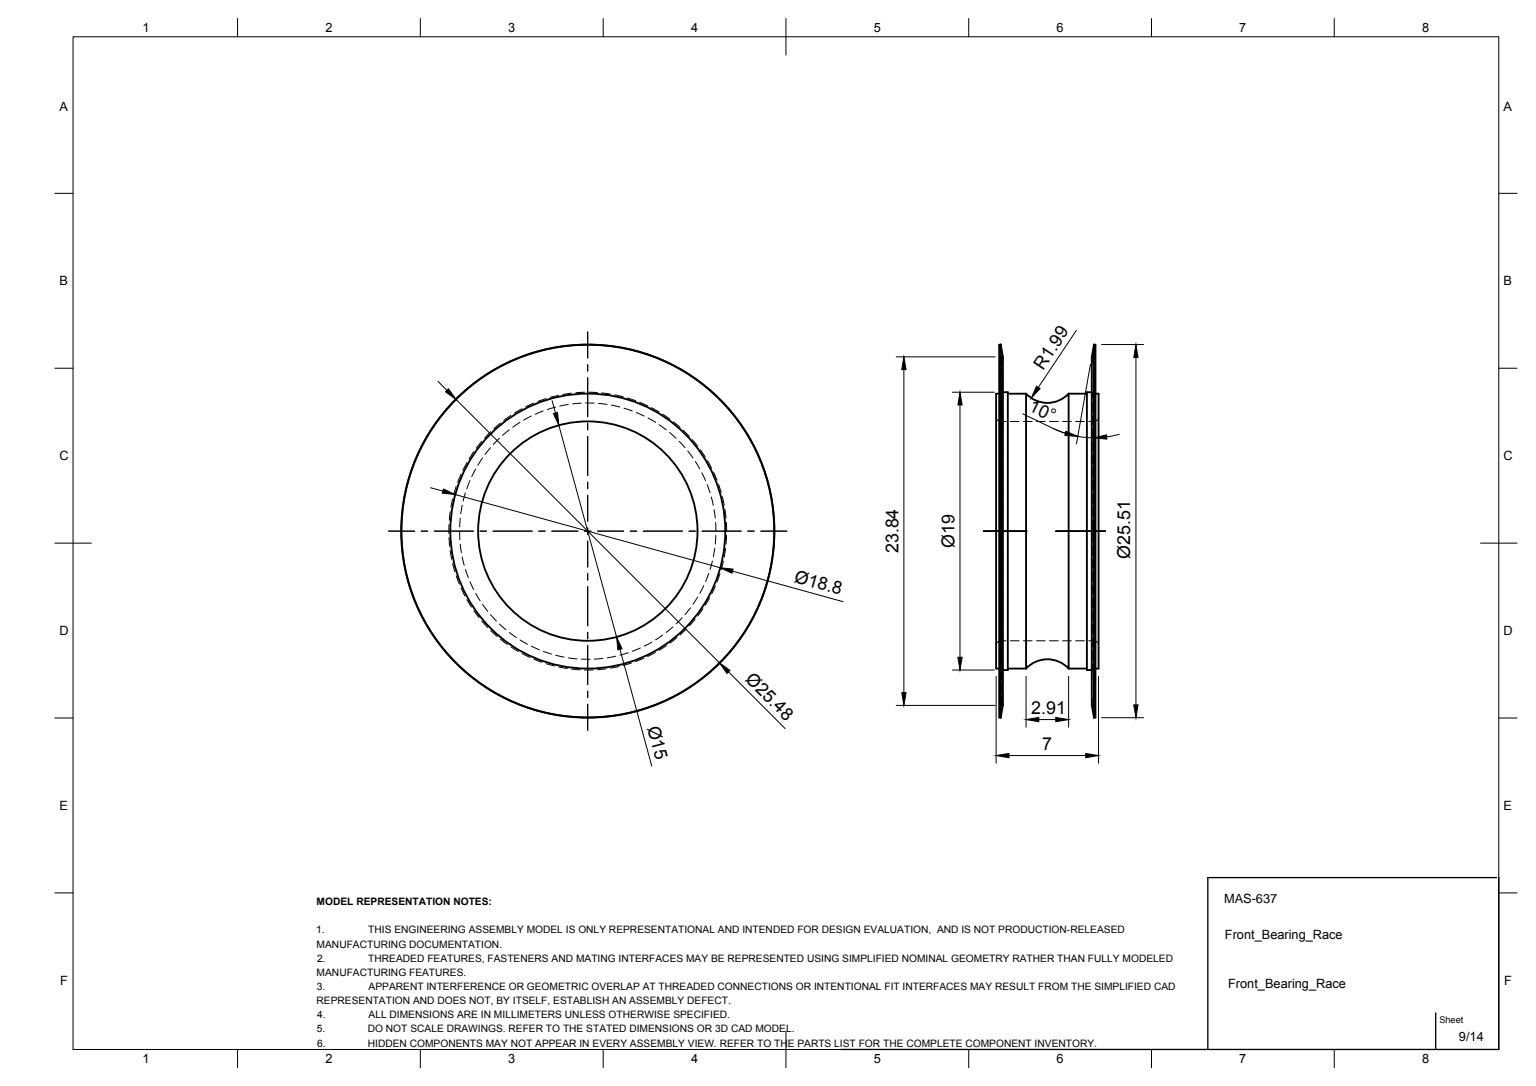
ISO-10303-21;
HEADER;
FILE_DESCRIPTION((''),'2;1');
FILE_NAME('Front_Bearing_Race.step','2026-10-09T10:11:57-07:00',(''),(''),'','','');
FILE_SCHEMA (('AUTOMOTIVE_DESIGN { 1 0 10303 214 3 1 1 }'));
ENDSEC;
DATA;
#10=MECHANICAL_DESIGN_GEOMETRIC_PRESENTATION_REPRESENTATION('',(#132),#13510);
#102=SHAPE_REPRESENTATION_RELATIONSHIP('SRR','None',#13572,#117) ;
#117=ADVANCED_BREP_SHAPE_REPRESENTATION('',(#164),#13504) ;
#132=STYLED_ITEM('',(#13650),#164) ;
#164=MANIFOLD_SOLID_BREP('Body1',#7381) ;
#246=FACE_BOUND('',#1504,.T.) ;
#247=FACE_BOUND('',#1515,.T.) ;
#248=FACE_BOUND('',#1519,.T.) ;
#249=FACE_BOUND('',#1523,.T.) ;
#250=FACE_BOUND('',#1525,.T.) ;
#251=FACE_BOUND('',#1534,.T.) ;
#252=FACE_BOUND('',#1542,.T.) ;
#253=FACE_BOUND('',#1546,.T.) ;
#454=PLANE('',#8257) ;
#455=PLANE('',#8281) ;
#456=PLANE('',#8288) ;
#457=PLANE('',#8296) ;
#458=PLANE('',#8298) ;
#459=PLANE('',#8318) ;
#460=PLANE('',#8333) ;
#461=PLANE('',#8340) ;
#501=TOROIDAL_SURFACE('',#8253,9.55,0.15) ;
#502=TOROIDAL_SURFACE('',#8259,11.3794692077,0.45) ;
#503=TOROIDAL_SURFACE('',#8264,11.8406976294,0.349999999988) ;
#504=TOROIDAL_SURFACE('',#8273,11.8406976294,0.45) ;
#505=TOROIDAL_SURFACE('',#8278,11.3794692077,0.35) ;
#506=TOROIDAL_SURFACE('',#8283,9.55,0.05) ;
#507=TOROIDAL_SURFACE('',#8290,9.55,0.15) ;
#508=TOROIDAL_SURFACE('',#8300,11.3794692077,0.45) ;
#509=TOROIDAL_SURFACE('',#8303,7.8,0.3) ;
#510=TOROIDAL_SURFACE('',#8310,11.8406976294,0.349999999988) ;
#511=TOROIDAL_SURFACE('',#8313,7.8,0.3) ;
#512=TOROIDAL_SURFACE('',#8325,11.8406976294,0.45) ;
#513=TOROIDAL_SURFACE('',#8330,11.3794692077,0.35) ;
#514=TOROIDAL_SURFACE('',#8335,9.55,0.05) ;
#515=TOROIDAL_SURFACE('',#8344,10.75,1.985) ;
#644=CYLINDRICAL_SURFACE('',#8286,9.5) ;
#645=CYLINDRICAL_SURFACE('',#8294,9.4) ;
#646=CYLINDRICAL_SURFACE('',#8308,7.5) ;
#647=CYLINDRICAL_SURFACE('',#8322,9.4) ;
#648=CYLINDRICAL_SURFACE('',#8338,9.5) ;
#649=CYLINDRICAL_SURFACE('',#8342,9.4) ;
#650=CYLINDRICAL_SURFACE('',#8347,9.4) ;
#995=FACE_OUTER_BOUND('',#1502,.T.) ;
#996=FACE_OUTER_BOUND('',#1503,.T.) ;
#997=FACE_OUTER_BOUND('',#1505,.T.) ;
#998=FACE_OUTER_BOUND('',#1506,.T.) ;
#999=FACE_OUTER_BOUND('',#1507,.T.) ;
#1000=FACE_OUTER_BOUND('',#1508,.T.) ;
#1001=FACE_OUTER_BOUND('',#1509,.T.) ;
#1002=FACE_OUTER_BOUND('',#1510,.T.) ;
#1003=FACE_OUTER_BOUND('',#1511,.T.) ;
#1004=FACE_OUTER_BOUND('',#1512,.T.) ;
#1005=FACE_OUTER_BOUND('',#1513,.T.) ;
#1006=FACE_OUTER_BOUND('',#1514,.T.) ;
#1007=FACE_OUTER_BOUND('',#1516,.T.) ;
#1008=FACE_OUTER_BOUND('',#1517,.T.) ;
#1009=FACE_OUTER_BOUND('',#1518,.T.) ;
#1010=FACE_OUTER_BOUND('',#1520,.T.) ;
#1011=FACE_OUTER_BOUND('',#1521,.T.) ;
#1012=FACE_OUTER_BOUND('',#1522,.T.) ;
#1013=FACE_OUTER_BOUND('',#1524,.T.) ;
#1014=FACE_OUTER_BOUND('',#1526,.T.) ;
#1015=FACE_OUTER_BOUND('',#1527,.T.) ;
#1016=FACE_OUTER_BOUND('',#1528,.T.) ;
#1017=FACE_OUTER_BOUND('',#1529,.T.) ;
#1018=FACE_OUTER_BOUND('',#1530,.T.) ;
#1019=FACE_OUTER_BOUND('',#1531,.T.) ;
#1020=FACE_OUTER_BOUND('',#1532,.T.) ;
#1021=FACE_OUTER_BOUND('',#1533,.T.) ;
#1022=FACE_OUTER_BOUND('',#1535,.T.) ;
#1023=FACE_OUTER_BOUND('',#1536,.T.) ;
#1024=FACE_OUTER_BOUND('',#1537,.T.) ;
#1025=FACE_OUTER_BOUND('',#1538,.T.) ;
#1026=FACE_OUTER_BOUND('',#1539,.T.) ;
#1027=FACE_OUTER_BOUND('',#1540,.T.) ;
#1028=FACE_OUTER_BOUND('',#1541,.T.) ;
#1029=FACE_OUTER_BOUND('',#1543,.T.) ;
#1030=FACE_OUTER_BOUND('',#1544,.T.) ;
#1031=FACE_OUTER_BOUND('',#1545,.T.) ;
#1032=FACE_OUTER_BOUND('',#1547,.T.) ;
#1033=FACE_OUTER_BOUND('',#1548,.T.) ;
#1034=FACE_OUTER_BOUND('',#1549,.T.) ;
#1502=EDGE_LOOP('',(#6440,#6441,#6442,#6443)) ;
#1503=EDGE_LOOP('',(#6444)) ;
#1504=EDGE_LOOP('',(#6445)) ;
#1505=EDGE_LOOP('',(#6446,#6447,#6448,#6449)) ;
#1506=EDGE_LOOP('',(#6450,#6451,#6452,#6453)) ;
#1507=EDGE_LOOP('',(#6454,#6455,#6456,#6457)) ;
#1508=EDGE_LOOP('',(#6458,#6459,#6460,#6461)) ;
#1509=EDGE_LOOP('',(#6462,#6463,#6464,#6465)) ;
#1510=EDGE_LOOP('',(#6466,#6467,#6468,#6469)) ;
#1511=EDGE_LOOP('',(#6470,#6471,#6472,#6473)) ;
#1512=EDGE_LOOP('',(#6474,#6475,#6476,#6477)) ;
#1513=EDGE_LOOP('',(#6478,#6479,#6480,#6481)) ;
#1514=EDGE_LOOP('',(#6482)) ;
#1515=EDGE_LOOP('',(#6483)) ;
#1516=EDGE_LOOP('',(#6484,#6485,#6486,#6487)) ;
#1517=EDGE_LOOP('',(#6488,#6489,#6490,#6491)) ;
#1518=EDGE_LOOP('',(#6492)) ;
#1519=EDGE_LOOP('',(#6493)) ;
#1520=EDGE_LOOP('',(#6494,#6495,#6496,#6497)) ;
#1521=EDGE_LOOP('',(#6498,#6499,#6500,#6501)) ;
#1522=EDGE_LOOP('',(#6502)) ;
#1523=EDGE_LOOP('',(#6503)) ;
#1524=EDGE_LOOP('',(#6504)) ;
#1525=EDGE_LOOP('',(#6505)) ;
#1526=EDGE_LOOP('',(#6506,#6507,#6508,#6509)) ;
#1527=EDGE_LOOP('',(#6510,#6511,#6512,#6513)) ;
#1528=EDGE_LOOP('',(#6514,#6515,#6516,#6517)) ;
#1529=EDGE_LOOP('',(#6518,#6519,#6520,#6521)) ;
#1530=EDGE_LOOP('',(#6522,#6523,#6524,#6525)) ;
#1531=EDGE_LOOP('',(#6526,#6527,#6528,#6529)) ;
#1532=EDGE_LOOP('',(#6530,#6531,#6532,#6533)) ;
#1533=EDGE_LOOP('',(#6534)) ;
#1534=EDGE_LOOP('',(#6535)) ;
#1535=EDGE_LOOP('',(#6536,#6537,#6538,#6539)) ;
#1536=EDGE_LOOP('',(#6540,#6541,#6542,#6543)) ;
#1537=EDGE_LOOP('',(#6544,#6545,#6546,#6547)) ;
#1538=EDGE_LOOP('',(#6548,#6549,#6550,#6551)) ;
#1539=EDGE_LOOP('',(#6552,#6553,#6554,#6555)) ;
#1540=EDGE_LOOP('',(#6556,#6557,#6558,#6559)) ;
#1541=EDGE_LOOP('',(#6560)) ;
#1542=EDGE_LOOP('',(#6561)) ;
#1543=EDGE_LOOP('',(#6562,#6563,#6564,#6565)) ;
#1544=EDGE_LOOP('',(#6566,#6567,#6568,#6569)) ;
#1545=EDGE_LOOP('',(#6570)) ;
#1546=EDGE_LOOP('',(#6571)) ;
#1547=EDGE_LOOP('',(#6572,#6573,#6574,#6575)) ;
#1548=EDGE_LOOP('',(#6576,#6577,#6578,#6579)) ;
#1549=EDGE_LOOP('',(#6580,#6581,#6582,#6583)) ;
#2095=LINE('',#12985,#2589) ;
#2096=LINE('',#12992,#2590) ;
#2097=LINE('',#12997,#2591) ;
#2098=LINE('',#13000,#2592) ;
#2099=LINE('',#13009,#2593) ;
#2100=LINE('',#13023,#2594) ;
#2101=LINE('',#13036,#2595) ;
#2102=LINE('',#13055,#2596) ;
#2103=LINE('',#13058,#2597) ;
#2104=LINE('',#13070,#2598) ;
#2105=LINE('',#13078,#2599) ;
#2106=LINE('',#13080,#2600) ;
#2107=LINE('',#13083,#2601) ;
#2108=LINE('',#13092,#2602) ;
#2109=LINE('',#13107,#2603) ;
#2110=LINE('',#13114,#2604) ;
#2111=LINE('',#13120,#2605) ;
#2589=VECTOR('',#10401,11.5333782722) ;
#2590=VECTOR('',#10410,11.9014744916) ;
#2591=VECTOR('',#10417,12.7397983664) ;
#2592=VECTOR('',#10420,11.9188393094) ;
#2593=VECTOR('',#10433,11.4991762579) ;
#2594=VECTOR('',#10452,9.5) ;
#2595=VECTOR('',#10469,9.4) ;
#2596=VECTOR('',#10496,11.5333782722) ;
#2597=VECTOR('',#10499,7.5) ;
#2598=VECTOR('',#10516,11.9014744916) ;
#2599=VECTOR('',#10527,12.7397983664) ;
#2600=VECTOR('',#10530,9.4) ;
#2601=VECTOR('',#10533,11.9188393094) ;
#2602=VECTOR('',#10546,11.4991762579) ;
#2603=VECTOR('',#10567,9.5) ;
#2604=VECTOR('',#10576,9.4) ;
#2605=VECTOR('',#10585,9.4) ;
#2976=CIRCLE('',#8254,9.4) ;
#2977=CIRCLE('',#8255,0.15) ;
#2978=CIRCLE('',#8256,9.55) ;
#2979=CIRCLE('',#8258,11.3794692077) ;
#2980=CIRCLE('',#8260,0.45) ;
#2981=CIRCLE('',#8261,11.5333782722) ;
#2982=CIRCLE('',#8263,11.7209905793) ;
#2983=CIRCLE('',#8265,0.349999999988) ;
#2984=CIRCLE('',#8266,11.9014744916) ;
#2985=CIRCLE('',#8268,12.7397983664) ;
#2986=CIRCLE('',#8270,12.7571631842) ;
#2987=CIRCLE('',#8272,11.9188393094) ;
#2988=CIRCLE('',#8274,0.45) ;
#2989=CIRCLE('',#8275,11.6867885649) ;
#2990=CIRCLE('',#8277,11.4991762579) ;
#2991=CIRCLE('',#8279,0.35) ;
#2992=CIRCLE('',#8280,11.3794692077) ;
#2993=CIRCLE('',#8282,9.55) ;
#2994=CIRCLE('',#8284,0.05) ;
#2995=CIRCLE('',#8285,9.5) ;
#2996=CIRCLE('',#8287,9.5) ;
#2997=CIRCLE('',#8289,9.4) ;
#2998=CIRCLE('',#8291,9.55) ;
#2999=CIRCLE('',#8292,0.15) ;
#3000=CIRCLE('',#8293,9.4) ;
#3001=CIRCLE('',#8295,9.4) ;
#3002=CIRCLE('',#8297,11.3794692077) ;
#3003=CIRCLE('',#8299,7.8) ;
#3004=CIRCLE('',#8301,11.5333782722) ;
#3005=CIRCLE('',#8302,0.45) ;
#3006=CIRCLE('',#8304,0.3) ;
#3007=CIRCLE('',#8305,7.5) ;
#3008=CIRCLE('',#8307,11.7209905793) ;
#3009=CIRCLE('',#8309,7.5) ;
#3010=CIRCLE('',#8311,11.9014744916) ;
#3011=CIRCLE('',#8312,0.349999999988) ;
#3012=CIRCLE('',#8314,0.3) ;
#3013=CIRCLE('',#8315,7.8) ;
#3014=CIRCLE('',#8317,12.7397983664) ;
#3015=CIRCLE('',#8319,9.4) ;
#3016=CIRCLE('',#8321,12.7571631842) ;
#3017=CIRCLE('',#8324,11.9188393094) ;
#3018=CIRCLE('',#8326,11.6867885649) ;
#3019=CIRCLE('',#8327,0.45) ;
#3020=CIRCLE('',#8329,11.4991762579) ;
#3021=CIRCLE('',#8331,11.3794692077) ;
#3022=CIRCLE('',#8332,0.35) ;
#3023=CIRCLE('',#8334,9.55) ;
#3024=CIRCLE('',#8336,9.5) ;
#3025=CIRCLE('',#8337,0.05) ;
#3026=CIRCLE('',#8339,9.5) ;
#3027=CIRCLE('',#8341,9.4) ;
#3028=CIRCLE('',#8343,9.4) ;
#3029=CIRCLE('',#8345,9.4) ;
#3030=CIRCLE('',#8346,1.985) ;
#3652=VERTEX_POINT('',#12970) ;
#3653=VERTEX_POINT('',#12972) ;
#3654=VERTEX_POINT('',#12976) ;
#3655=VERTEX_POINT('',#12979) ;
#3656=VERTEX_POINT('',#12983) ;
#3657=VERTEX_POINT('',#12987) ;
#3658=VERTEX_POINT('',#12991) ;
#3659=VERTEX_POINT('',#12995) ;
#3660=VERTEX_POINT('',#12999) ;
#3661=VERTEX_POINT('',#13003) ;
#3662=VERTEX_POINT('',#13007) ;
#3663=VERTEX_POINT('',#13011) ;
#3664=VERTEX_POINT('',#13015) ;
#3665=VERTEX_POINT('',#13018) ;
#3666=VERTEX_POINT('',#13022) ;
#3667=VERTEX_POINT('',#13026) ;
#3668=VERTEX_POINT('',#13029) ;
#3669=VERTEX_POINT('',#13031) ;
#3670=VERTEX_POINT('',#13035) ;
#3671=VERTEX_POINT('',#13039) ;
#3672=VERTEX_POINT('',#13042) ;
#3673=VERTEX_POINT('',#13045) ;
#3674=VERTEX_POINT('',#13049) ;
#3675=VERTEX_POINT('',#13053) ;
#3676=VERTEX_POINT('',#13057) ;
#3677=VERTEX_POINT('',#13061) ;
#3678=VERTEX_POINT('',#13065) ;
#3679=VERTEX_POINT('',#13069) ;
#3680=VERTEX_POINT('',#13073) ;
#3681=VERTEX_POINT('',#13076) ;
#3682=VERTEX_POINT('',#13082) ;
#3683=VERTEX_POINT('',#13086) ;
#3684=VERTEX_POINT('',#13090) ;
#3685=VERTEX_POINT('',#13094) ;
#3686=VERTEX_POINT('',#13098) ;
#3687=VERTEX_POINT('',#13101) ;
#3688=VERTEX_POINT('',#13105) ;
#3689=VERTEX_POINT('',#13109) ;
#3690=VERTEX_POINT('',#13112) ;
#3691=VERTEX_POINT('',#13116) ;
#4607=EDGE_CURVE('',#3652,#3652,#2976,.T.) ;
#4608=EDGE_CURVE('',#3652,#3653,#2977,.T.) ;
#4609=EDGE_CURVE('',#3653,#3653,#2978,.T.) ;
#4610=EDGE_CURVE('',#3654,#3654,#2979,.T.) ;
#4611=EDGE_CURVE('',#3654,#3655,#2980,.T.) ;
#4612=EDGE_CURVE('',#3655,#3655,#2981,.T.) ;
#4613=EDGE_CURVE('',#3656,#3656,#2982,.F.) ;
#4614=EDGE_CURVE('',#3656,#3655,#2095,.T.) ;
#4615=EDGE_CURVE('',#3656,#3657,#2983,.T.) ;
#4616=EDGE_CURVE('',#3657,#3657,#2984,.T.) ;
#4617=EDGE_CURVE('',#3657,#3658,#2096,.T.) ;
#4618=EDGE_CURVE('',#3658,#3658,#2985,.T.) ;
#4619=EDGE_CURVE('',#3659,#3659,#2986,.F.) ;
#4620=EDGE_CURVE('',#3659,#3658,#2097,.T.) ;
#4621=EDGE_CURVE('',#3659,#3660,#2098,.T.) ;
#4622=EDGE_CURVE('',#3660,#3660,#2987,.T.) ;
#4623=EDGE_CURVE('',#3660,#3661,#2988,.T.) ;
#4624=EDGE_CURVE('',#3661,#3661,#2989,.T.) ;
#4625=EDGE_CURVE('',#3662,#3662,#2990,.F.) ;
#4626=EDGE_CURVE('',#3662,#3661,#2099,.T.) ;
#4627=EDGE_CURVE('',#3662,#3663,#2991,.T.) ;
#4628=EDGE_CURVE('',#3663,#3663,#2992,.T.) ;
#4629=EDGE_CURVE('',#3664,#3664,#2993,.T.) ;
#4630=EDGE_CURVE('',#3664,#3665,#2994,.T.) ;
#4631=EDGE_CURVE('',#3665,#3665,#2995,.T.) ;
#4632=EDGE_CURVE('',#3665,#3666,#2100,.T.) ;
#4633=EDGE_CURVE('',#3666,#3666,#2996,.T.) ;
#4634=EDGE_CURVE('',#3667,#3667,#2997,.T.) ;
#4635=EDGE_CURVE('',#3668,#3668,#2998,.T.) ;
#4636=EDGE_CURVE('',#3668,#3669,#2999,.T.) ;
#4637=EDGE_CURVE('',#3669,#3669,#3000,.T.) ;
#4638=EDGE_CURVE('',#3669,#3670,#2101,.T.) ;
#4639=EDGE_CURVE('',#3670,#3670,#3001,.T.) ;
#4640=EDGE_CURVE('',#3671,#3671,#3002,.T.) ;
#4641=EDGE_CURVE('',#3672,#3672,#3003,.T.) ;
#4642=EDGE_CURVE('',#3673,#3673,#3004,.T.) ;
#4643=EDGE_CURVE('',#3673,#3671,#3005,.T.) ;
#4644=EDGE_CURVE('',#3672,#3674,#3006,.T.) ;
#4645=EDGE_CURVE('',#3674,#3674,#3007,.T.) ;
#4646=EDGE_CURVE('',#3675,#3675,#3008,.T.) ;
#4647=EDGE_CURVE('',#3675,#3673,#2102,.T.) ;
#4648=EDGE_CURVE('',#3674,#3676,#2103,.T.) ;
#4649=EDGE_CURVE('',#3676,#3676,#3009,.T.) ;
#4650=EDGE_CURVE('',#3677,#3677,#3010,.T.) ;
#4651=EDGE_CURVE('',#3677,#3675,#3011,.T.) ;
#4652=EDGE_CURVE('',#3676,#3678,#3012,.T.) ;
#4653=EDGE_CURVE('',#3678,#3678,#3013,.T.) ;
#4654=EDGE_CURVE('',#3677,#3679,#2104,.T.) ;
#4655=EDGE_CURVE('',#3679,#3679,#3014,.F.) ;
#4656=EDGE_CURVE('',#3680,#3680,#3015,.T.) ;
#4657=EDGE_CURVE('',#3681,#3681,#3016,.T.) ;
#4658=EDGE_CURVE('',#3681,#3679,#2105,.T.) ;
#4659=EDGE_CURVE('',#3680,#3652,#2106,.T.) ;
#4660=EDGE_CURVE('',#3681,#3682,#2107,.T.) ;
#4661=EDGE_CURVE('',#3682,#3682,#3017,.F.) ;
#4662=EDGE_CURVE('',#3683,#3683,#3018,.T.) ;
#4663=EDGE_CURVE('',#3683,#3682,#3019,.T.) ;
#4664=EDGE_CURVE('',#3684,#3684,#3020,.T.) ;
#4665=EDGE_CURVE('',#3684,#3683,#2108,.T.) ;
#4666=EDGE_CURVE('',#3685,#3685,#3021,.T.) ;
#4667=EDGE_CURVE('',#3685,#3684,#3022,.T.) ;
#4668=EDGE_CURVE('',#3686,#3686,#3023,.T.) ;
#4669=EDGE_CURVE('',#3687,#3687,#3024,.T.) ;
#4670=EDGE_CURVE('',#3687,#3686,#3025,.T.) ;
#4671=EDGE_CURVE('',#3688,#3688,#3026,.T.) ;
#4672=EDGE_CURVE('',#3688,#3687,#2109,.T.) ;
#4673=EDGE_CURVE('',#3689,#3689,#3027,.T.) ;
#4674=EDGE_CURVE('',#3690,#3690,#3028,.T.) ;
#4675=EDGE_CURVE('',#3690,#3689,#2110,.T.) ;
#4676=EDGE_CURVE('',#3691,#3691,#3029,.T.) ;
#4677=EDGE_CURVE('',#3691,#3690,#3030,.T.) ;
#4678=EDGE_CURVE('',#3667,#3691,#2111,.T.) ;
#6440=ORIENTED_EDGE('',*,*,#4607,.F.) ;
#6441=ORIENTED_EDGE('',*,*,#4608,.T.) ;
#6442=ORIENTED_EDGE('',*,*,#4609,.T.) ;
#6443=ORIENTED_EDGE('',*,*,#4608,.F.) ;
#6444=ORIENTED_EDGE('',*,*,#4610,.T.) ;
#6445=ORIENTED_EDGE('',*,*,#4609,.F.) ;
#6446=ORIENTED_EDGE('',*,*,#4610,.F.) ;
#6447=ORIENTED_EDGE('',*,*,#4611,.T.) ;
#6448=ORIENTED_EDGE('',*,*,#4612,.T.) ;
#6449=ORIENTED_EDGE('',*,*,#4611,.F.) ;
#6450=ORIENTED_EDGE('',*,*,#4613,.T.) ;
#6451=ORIENTED_EDGE('',*,*,#4614,.T.) ;
#6452=ORIENTED_EDGE('',*,*,#4612,.F.) ;
#6453=ORIENTED_EDGE('',*,*,#4614,.F.) ;
#6454=ORIENTED_EDGE('',*,*,#4613,.F.) ;
#6455=ORIENTED_EDGE('',*,*,#4615,.T.) ;
#6456=ORIENTED_EDGE('',*,*,#4616,.T.) ;
#6457=ORIENTED_EDGE('',*,*,#4615,.F.) ;
#6458=ORIENTED_EDGE('',*,*,#4616,.F.) ;
#6459=ORIENTED_EDGE('',*,*,#4617,.T.) ;
#6460=ORIENTED_EDGE('',*,*,#4618,.T.) ;
#6461=ORIENTED_EDGE('',*,*,#4617,.F.) ;
#6462=ORIENTED_EDGE('',*,*,#4619,.T.) ;
#6463=ORIENTED_EDGE('',*,*,#4620,.T.) ;
#6464=ORIENTED_EDGE('',*,*,#4618,.F.) ;
#6465=ORIENTED_EDGE('',*,*,#4620,.F.) ;
#6466=ORIENTED_EDGE('',*,*,#4619,.F.) ;
#6467=ORIENTED_EDGE('',*,*,#4621,.T.) ;
#6468=ORIENTED_EDGE('',*,*,#4622,.T.) ;
#6469=ORIENTED_EDGE('',*,*,#4621,.F.) ;
#6470=ORIENTED_EDGE('',*,*,#4622,.F.) ;
#6471=ORIENTED_EDGE('',*,*,#4623,.T.) ;
#6472=ORIENTED_EDGE('',*,*,#4624,.T.) ;
#6473=ORIENTED_EDGE('',*,*,#4623,.F.) ;
#6474=ORIENTED_EDGE('',*,*,#4625,.T.) ;
#6475=ORIENTED_EDGE('',*,*,#4626,.T.) ;
#6476=ORIENTED_EDGE('',*,*,#4624,.F.) ;
#6477=ORIENTED_EDGE('',*,*,#4626,.F.) ;
#6478=ORIENTED_EDGE('',*,*,#4625,.F.) ;
#6479=ORIENTED_EDGE('',*,*,#4627,.T.) ;
#6480=ORIENTED_EDGE('',*,*,#4628,.T.) ;
#6481=ORIENTED_EDGE('',*,*,#4627,.F.) ;
#6482=ORIENTED_EDGE('',*,*,#4628,.F.) ;
#6483=ORIENTED_EDGE('',*,*,#4629,.T.) ;
#6484=ORIENTED_EDGE('',*,*,#4629,.F.) ;
#6485=ORIENTED_EDGE('',*,*,#4630,.T.) ;
#6486=ORIENTED_EDGE('',*,*,#4631,.T.) ;
#6487=ORIENTED_EDGE('',*,*,#4630,.F.) ;
#6488=ORIENTED_EDGE('',*,*,#4631,.F.) ;
#6489=ORIENTED_EDGE('',*,*,#4632,.T.) ;
#6490=ORIENTED_EDGE('',*,*,#4633,.T.) ;
#6491=ORIENTED_EDGE('',*,*,#4632,.F.) ;
#6492=ORIENTED_EDGE('',*,*,#4633,.F.) ;
#6493=ORIENTED_EDGE('',*,*,#4634,.T.) ;
#6494=ORIENTED_EDGE('',*,*,#4635,.F.) ;
#6495=ORIENTED_EDGE('',*,*,#4636,.T.) ;
#6496=ORIENTED_EDGE('',*,*,#4637,.T.) ;
#6497=ORIENTED_EDGE('',*,*,#4636,.F.) ;
#6498=ORIENTED_EDGE('',*,*,#4637,.F.) ;
#6499=ORIENTED_EDGE('',*,*,#4638,.T.) ;
#6500=ORIENTED_EDGE('',*,*,#4639,.T.) ;
#6501=ORIENTED_EDGE('',*,*,#4638,.F.) ;
#6502=ORIENTED_EDGE('',*,*,#4640,.F.) ;
#6503=ORIENTED_EDGE('',*,*,#4635,.T.) ;
#6504=ORIENTED_EDGE('',*,*,#4639,.F.) ;
#6505=ORIENTED_EDGE('',*,*,#4641,.T.) ;
#6506=ORIENTED_EDGE('',*,*,#4642,.F.) ;
#6507=ORIENTED_EDGE('',*,*,#4643,.T.) ;
#6508=ORIENTED_EDGE('',*,*,#4640,.T.) ;
#6509=ORIENTED_EDGE('',*,*,#4643,.F.) ;
#6510=ORIENTED_EDGE('',*,*,#4641,.F.) ;
#6511=ORIENTED_EDGE('',*,*,#4644,.T.) ;
#6512=ORIENTED_EDGE('',*,*,#4645,.T.) ;
#6513=ORIENTED_EDGE('',*,*,#4644,.F.) ;
#6514=ORIENTED_EDGE('',*,*,#4646,.F.) ;
#6515=ORIENTED_EDGE('',*,*,#4647,.T.) ;
#6516=ORIENTED_EDGE('',*,*,#4642,.T.) ;
#6517=ORIENTED_EDGE('',*,*,#4647,.F.) ;
#6518=ORIENTED_EDGE('',*,*,#4645,.F.) ;
#6519=ORIENTED_EDGE('',*,*,#4648,.T.) ;
#6520=ORIENTED_EDGE('',*,*,#4649,.T.) ;
#6521=ORIENTED_EDGE('',*,*,#4648,.F.) ;
#6522=ORIENTED_EDGE('',*,*,#4650,.F.) ;
#6523=ORIENTED_EDGE('',*,*,#4651,.T.) ;
#6524=ORIENTED_EDGE('',*,*,#4646,.T.) ;
#6525=ORIENTED_EDGE('',*,*,#4651,.F.) ;
#6526=ORIENTED_EDGE('',*,*,#4649,.F.) ;
#6527=ORIENTED_EDGE('',*,*,#4652,.T.) ;
#6528=ORIENTED_EDGE('',*,*,#4653,.T.) ;
#6529=ORIENTED_EDGE('',*,*,#4652,.F.) ;
#6530=ORIENTED_EDGE('',*,*,#4650,.T.) ;
#6531=ORIENTED_EDGE('',*,*,#4654,.T.) ;
#6532=ORIENTED_EDGE('',*,*,#4655,.F.) ;
#6533=ORIENTED_EDGE('',*,*,#4654,.F.) ;
#6534=ORIENTED_EDGE('',*,*,#4656,.T.) ;
#6535=ORIENTED_EDGE('',*,*,#4653,.F.) ;
#6536=ORIENTED_EDGE('',*,*,#4657,.F.) ;
#6537=ORIENTED_EDGE('',*,*,#4658,.T.) ;
#6538=ORIENTED_EDGE('',*,*,#4655,.T.) ;
#6539=ORIENTED_EDGE('',*,*,#4658,.F.) ;
#6540=ORIENTED_EDGE('',*,*,#4656,.F.) ;
#6541=ORIENTED_EDGE('',*,*,#4659,.T.) ;
#6542=ORIENTED_EDGE('',*,*,#4607,.T.) ;
#6543=ORIENTED_EDGE('',*,*,#4659,.F.) ;
#6544=ORIENTED_EDGE('',*,*,#4657,.T.) ;
#6545=ORIENTED_EDGE('',*,*,#4660,.T.) ;
#6546=ORIENTED_EDGE('',*,*,#4661,.F.) ;
#6547=ORIENTED_EDGE('',*,*,#4660,.F.) ;
#6548=ORIENTED_EDGE('',*,*,#4662,.F.) ;
#6549=ORIENTED_EDGE('',*,*,#4663,.T.) ;
#6550=ORIENTED_EDGE('',*,*,#4661,.T.) ;
#6551=ORIENTED_EDGE('',*,*,#4663,.F.) ;
#6552=ORIENTED_EDGE('',*,*,#4664,.F.) ;
#6553=ORIENTED_EDGE('',*,*,#4665,.T.) ;
#6554=ORIENTED_EDGE('',*,*,#4662,.T.) ;
#6555=ORIENTED_EDGE('',*,*,#4665,.F.) ;
#6556=ORIENTED_EDGE('',*,*,#4666,.F.) ;
#6557=ORIENTED_EDGE('',*,*,#4667,.T.) ;
#6558=ORIENTED_EDGE('',*,*,#4664,.T.) ;
#6559=ORIENTED_EDGE('',*,*,#4667,.F.) ;
#6560=ORIENTED_EDGE('',*,*,#4666,.T.) ;
#6561=ORIENTED_EDGE('',*,*,#4668,.F.) ;
#6562=ORIENTED_EDGE('',*,*,#4669,.F.) ;
#6563=ORIENTED_EDGE('',*,*,#4670,.T.) ;
#6564=ORIENTED_EDGE('',*,*,#4668,.T.) ;
#6565=ORIENTED_EDGE('',*,*,#4670,.F.) ;
#6566=ORIENTED_EDGE('',*,*,#4671,.F.) ;
#6567=ORIENTED_EDGE('',*,*,#4672,.T.) ;
#6568=ORIENTED_EDGE('',*,*,#4669,.T.) ;
#6569=ORIENTED_EDGE('',*,*,#4672,.F.) ;
#6570=ORIENTED_EDGE('',*,*,#4671,.T.) ;
#6571=ORIENTED_EDGE('',*,*,#4673,.F.) ;
#6572=ORIENTED_EDGE('',*,*,#4674,.F.) ;
#6573=ORIENTED_EDGE('',*,*,#4675,.T.) ;
#6574=ORIENTED_EDGE('',*,*,#4673,.T.) ;
#6575=ORIENTED_EDGE('',*,*,#4675,.F.) ;
#6576=ORIENTED_EDGE('',*,*,#4676,.F.) ;
#6577=ORIENTED_EDGE('',*,*,#4677,.T.) ;
#6578=ORIENTED_EDGE('',*,*,#4674,.T.) ;
#6579=ORIENTED_EDGE('',*,*,#4677,.F.) ;
#6580=ORIENTED_EDGE('',*,*,#4634,.F.) ;
#6581=ORIENTED_EDGE('',*,*,#4678,.T.) ;
#6582=ORIENTED_EDGE('',*,*,#4676,.T.) ;
#6583=ORIENTED_EDGE('',*,*,#4678,.F.) ;
#6894=CONICAL_SURFACE('',#8262,11.5333782722,1.2217304764) ;
#6895=CONICAL_SURFACE('',#8267,11.9014744916,1.3962634016) ;
#6896=CONICAL_SURFACE('',#8269,12.7397983664,0.174532925199) ;
#6897=CONICAL_SURFACE('',#8271,11.9188393094,1.3962634016) ;
#6898=CONICAL_SURFACE('',#8276,11.4991762579,1.2217304764) ;
#6899=CONICAL_SURFACE('',#8306,11.5333782722,1.2217304764) ;
#6900=CONICAL_SURFACE('',#8316,11.9014744916,1.3962634016) ;
#6901=CONICAL_SURFACE('',#8320,12.7397983664,0.174532925199) ;
#6902=CONICAL_SURFACE('',#8323,11.9188393094,1.3962634016) ;
#6903=CONICAL_SURFACE('',#8328,11.4991762579,1.2217304764) ;
#7245=ADVANCED_FACE('',(#995),#501,.T.) ;
#7246=ADVANCED_FACE('',(#996,#246),#454,.T.) ;
#7247=ADVANCED_FACE('',(#997),#502,.T.) ;
#7248=ADVANCED_FACE('',(#998),#6894,.T.) ;
#7249=ADVANCED_FACE('',(#999),#503,.F.) ;
#7250=ADVANCED_FACE('',(#1000),#6895,.F.) ;
#7251=ADVANCED_FACE('',(#1001),#6896,.T.) ;
#7252=ADVANCED_FACE('',(#1002),#6897,.T.) ;
#7253=ADVANCED_FACE('',(#1003),#504,.T.) ;
#7254=ADVANCED_FACE('',(#1004),#6898,.F.) ;
#7255=ADVANCED_FACE('',(#1005),#505,.F.) ;
#7256=ADVANCED_FACE('',(#1006,#247),#455,.F.) ;
#7257=ADVANCED_FACE('',(#1007),#506,.F.) ;
#7258=ADVANCED_FACE('',(#1008),#644,.T.) ;
#7259=ADVANCED_FACE('',(#1009,#248),#456,.F.) ;
#7260=ADVANCED_FACE('',(#1010),#507,.T.) ;
#7261=ADVANCED_FACE('',(#1011),#645,.T.) ;
#7262=ADVANCED_FACE('',(#1012,#249),#457,.F.) ;
#7263=ADVANCED_FACE('',(#1013,#250),#458,.F.) ;
#7264=ADVANCED_FACE('',(#1014),#508,.T.) ;
#7265=ADVANCED_FACE('',(#1015),#509,.T.) ;
#7266=ADVANCED_FACE('',(#1016),#6899,.T.) ;
#7267=ADVANCED_FACE('',(#1017),#646,.F.) ;
#7268=ADVANCED_FACE('',(#1018),#510,.F.) ;
#7269=ADVANCED_FACE('',(#1019),#511,.T.) ;
#7270=ADVANCED_FACE('',(#1020),#6900,.F.) ;
#7271=ADVANCED_FACE('',(#1021,#251),#459,.T.) ;
#7272=ADVANCED_FACE('',(#1022),#6901,.T.) ;
#7273=ADVANCED_FACE('',(#1023),#647,.T.) ;
#7274=ADVANCED_FACE('',(#1024),#6902,.T.) ;
#7275=ADVANCED_FACE('',(#1025),#512,.T.) ;
#7276=ADVANCED_FACE('',(#1026),#6903,.F.) ;
#7277=ADVANCED_FACE('',(#1027),#513,.F.) ;
#7278=ADVANCED_FACE('',(#1028,#252),#460,.T.) ;
#7279=ADVANCED_FACE('',(#1029),#514,.F.) ;
#7280=ADVANCED_FACE('',(#1030),#648,.T.) ;
#7281=ADVANCED_FACE('',(#1031,#253),#461,.T.) ;
#7282=ADVANCED_FACE('',(#1032),#649,.T.) ;
#7283=ADVANCED_FACE('',(#1033),#515,.F.) ;
#7284=ADVANCED_FACE('',(#1034),#650,.T.) ;
#7381=CLOSED_SHELL('',(#7245,#7246,#7247,#7248,#7249,#7250,#7251,#7252,
#7253,#7254,#7255,#7256,#7257,#7258,#7259,#7260,#7261,#7262,#7263,#7264,
#7265,#7266,#7267,#7268,#7269,#7270,#7271,#7272,#7273,#7274,#7275,#7276,
#7277,#7278,#7279,#7280,#7281,#7282,#7283,#7284)) ;
#8252=AXIS2_PLACEMENT_3D('',#12968,#10377,#10378) ;
#8253=AXIS2_PLACEMENT_3D('',#12969,#10379,#10380) ;
#8254=AXIS2_PLACEMENT_3D('',#12971,#10381,#10382) ;
#8255=AXIS2_PLACEMENT_3D('',#12973,#10383,#10384) ;
#8256=AXIS2_PLACEMENT_3D('',#12974,#10385,#10386) ;
#8257=AXIS2_PLACEMENT_3D('',#12975,#10387,#10388) ;
#8258=AXIS2_PLACEMENT_3D('',#12977,#10389,#10390) ;
#8259=AXIS2_PLACEMENT_3D('',#12978,#10391,#10392) ;
#8260=AXIS2_PLACEMENT_3D('',#12980,#10393,#10394) ;
#8261=AXIS2_PLACEMENT_3D('',#12981,#10395,#10396) ;
#8262=AXIS2_PLACEMENT_3D('',#12982,#10397,#10398) ;
#8263=AXIS2_PLACEMENT_3D('',#12984,#10399,#10400) ;
#8264=AXIS2_PLACEMENT_3D('',#12986,#10402,#10403) ;
#8265=AXIS2_PLACEMENT_3D('',#12988,#10404,#10405) ;
#8266=AXIS2_PLACEMENT_3D('',#12989,#10406,#10407) ;
#8267=AXIS2_PLACEMENT_3D('',#12990,#10408,#10409) ;
#8268=AXIS2_PLACEMENT_3D('',#12993,#10411,#10412) ;
#8269=AXIS2_PLACEMENT_3D('',#12994,#10413,#10414) ;
#8270=AXIS2_PLACEMENT_3D('',#12996,#10415,#10416) ;
#8271=AXIS2_PLACEMENT_3D('',#12998,#10418,#10419) ;
#8272=AXIS2_PLACEMENT_3D('',#13001,#10421,#10422) ;
#8273=AXIS2_PLACEMENT_3D('',#13002,#10423,#10424) ;
#8274=AXIS2_PLACEMENT_3D('',#13004,#10425,#10426) ;
#8275=AXIS2_PLACEMENT_3D('',#13005,#10427,#10428) ;
#8276=AXIS2_PLACEMENT_3D('',#13006,#10429,#10430) ;
#8277=AXIS2_PLACEMENT_3D('',#13008,#10431,#10432) ;
#8278=AXIS2_PLACEMENT_3D('',#13010,#10434,#10435) ;
#8279=AXIS2_PLACEMENT_3D('',#13012,#10436,#10437) ;
#8280=AXIS2_PLACEMENT_3D('',#13013,#10438,#10439) ;
#8281=AXIS2_PLACEMENT_3D('',#13014,#10440,#10441) ;
#8282=AXIS2_PLACEMENT_3D('',#13016,#10442,#10443) ;
#8283=AXIS2_PLACEMENT_3D('',#13017,#10444,#10445) ;
#8284=AXIS2_PLACEMENT_3D('',#13019,#10446,#10447) ;
#8285=AXIS2_PLACEMENT_3D('',#13020,#10448,#10449) ;
#8286=AXIS2_PLACEMENT_3D('',#13021,#10450,#10451) ;
#8287=AXIS2_PLACEMENT_3D('',#13024,#10453,#10454) ;
#8288=AXIS2_PLACEMENT_3D('',#13025,#10455,#10456) ;
#8289=AXIS2_PLACEMENT_3D('',#13027,#10457,#10458) ;
#8290=AXIS2_PLACEMENT_3D('',#13028,#10459,#10460) ;
#8291=AXIS2_PLACEMENT_3D('',#13030,#10461,#10462) ;
#8292=AXIS2_PLACEMENT_3D('',#13032,#10463,#10464) ;
#8293=AXIS2_PLACEMENT_3D('',#13033,#10465,#10466) ;
#8294=AXIS2_PLACEMENT_3D('',#13034,#10467,#10468) ;
#8295=AXIS2_PLACEMENT_3D('',#13037,#10470,#10471) ;
#8296=AXIS2_PLACEMENT_3D('',#13038,#10472,#10473) ;
#8297=AXIS2_PLACEMENT_3D('',#13040,#10474,#10475) ;
#8298=AXIS2_PLACEMENT_3D('',#13041,#10476,#10477) ;
#8299=AXIS2_PLACEMENT_3D('',#13043,#10478,#10479) ;
#8300=AXIS2_PLACEMENT_3D('',#13044,#10480,#10481) ;
#8301=AXIS2_PLACEMENT_3D('',#13046,#10482,#10483) ;
#8302=AXIS2_PLACEMENT_3D('',#13047,#10484,#10485) ;
#8303=AXIS2_PLACEMENT_3D('',#13048,#10486,#10487) ;
#8304=AXIS2_PLACEMENT_3D('',#13050,#10488,#10489) ;
#8305=AXIS2_PLACEMENT_3D('',#13051,#10490,#10491) ;
#8306=AXIS2_PLACEMENT_3D('',#13052,#10492,#10493) ;
#8307=AXIS2_PLACEMENT_3D('',#13054,#10494,#10495) ;
#8308=AXIS2_PLACEMENT_3D('',#13056,#10497,#10498) ;
#8309=AXIS2_PLACEMENT_3D('',#13059,#10500,#10501) ;
#8310=AXIS2_PLACEMENT_3D('',#13060,#10502,#10503) ;
#8311=AXIS2_PLACEMENT_3D('',#13062,#10504,#10505) ;
#8312=AXIS2_PLACEMENT_3D('',#13063,#10506,#10507) ;
#8313=AXIS2_PLACEMENT_3D('',#13064,#10508,#10509) ;
#8314=AXIS2_PLACEMENT_3D('',#13066,#10510,#10511) ;
#8315=AXIS2_PLACEMENT_3D('',#13067,#10512,#10513) ;
#8316=AXIS2_PLACEMENT_3D('',#13068,#10514,#10515) ;
#8317=AXIS2_PLACEMENT_3D('',#13071,#10517,#10518) ;
#8318=AXIS2_PLACEMENT_3D('',#13072,#10519,#10520) ;
#8319=AXIS2_PLACEMENT_3D('',#13074,#10521,#10522) ;
#8320=AXIS2_PLACEMENT_3D('',#13075,#10523,#10524) ;
#8321=AXIS2_PLACEMENT_3D('',#13077,#10525,#10526) ;
#8322=AXIS2_PLACEMENT_3D('',#13079,#10528,#10529) ;
#8323=AXIS2_PLACEMENT_3D('',#13081,#10531,#10532) ;
#8324=AXIS2_PLACEMENT_3D('',#13084,#10534,#10535) ;
#8325=AXIS2_PLACEMENT_3D('',#13085,#10536,#10537) ;
#8326=AXIS2_PLACEMENT_3D('',#13087,#10538,#10539) ;
#8327=AXIS2_PLACEMENT_3D('',#13088,#10540,#10541) ;
#8328=AXIS2_PLACEMENT_3D('',#13089,#10542,#10543) ;
#8329=AXIS2_PLACEMENT_3D('',#13091,#10544,#10545) ;
#8330=AXIS2_PLACEMENT_3D('',#13093,#10547,#10548) ;
#8331=AXIS2_PLACEMENT_3D('',#13095,#10549,#10550) ;
#8332=AXIS2_PLACEMENT_3D('',#13096,#10551,#10552) ;
#8333=AXIS2_PLACEMENT_3D('',#13097,#10553,#10554) ;
#8334=AXIS2_PLACEMENT_3D('',#13099,#10555,#10556) ;
#8335=AXIS2_PLACEMENT_3D('',#13100,#10557,#10558) ;
#8336=AXIS2_PLACEMENT_3D('',#13102,#10559,#10560) ;
#8337=AXIS2_PLACEMENT_3D('',#13103,#10561,#10562) ;
#8338=AXIS2_PLACEMENT_3D('',#13104,#10563,#10564) ;
#8339=AXIS2_PLACEMENT_3D('',#13106,#10565,#10566) ;
#8340=AXIS2_PLACEMENT_3D('',#13108,#10568,#10569) ;
#8341=AXIS2_PLACEMENT_3D('',#13110,#10570,#10571) ;
#8342=AXIS2_PLACEMENT_3D('',#13111,#10572,#10573) ;
#8343=AXIS2_PLACEMENT_3D('',#13113,#10574,#10575) ;
#8344=AXIS2_PLACEMENT_3D('',#13115,#10577,#10578) ;
#8345=AXIS2_PLACEMENT_3D('',#13117,#10579,#10580) ;
#8346=AXIS2_PLACEMENT_3D('',#13118,#10581,#10582) ;
#8347=AXIS2_PLACEMENT_3D('',#13119,#10583,#10584) ;
#10377=DIRECTION('axis',(0.,0.,1.)) ;
#10378=DIRECTION('refdir',(1.,0.,0.)) ;
#10379=DIRECTION('center_axis',(0.,0.,-1.)) ;
#10380=DIRECTION('ref_axis',(0.877582561890372,-0.479425538604204,0.)) ;
#10381=DIRECTION('center_axis',(0.,0.,-1.)) ;
#10382=DIRECTION('ref_axis',(1.,0.,0.)) ;
#10383=DIRECTION('center_axis',(0.479425538604204,0.877582561890372,0.)) ;
#10384=DIRECTION('ref_axis',(-0.877582561890372,0.479425538604204,0.)) ;
#10385=DIRECTION('center_axis',(0.,0.,-1.)) ;
#10386=DIRECTION('ref_axis',(1.,0.,0.)) ;
#10387=DIRECTION('center_axis',(0.,0.,-1.)) ;
#10388=DIRECTION('ref_axis',(1.,0.,0.)) ;
#10389=DIRECTION('center_axis',(0.,0.,-1.)) ;
#10390=DIRECTION('ref_axis',(1.,0.,0.)) ;
#10391=DIRECTION('center_axis',(0.,0.,-1.)) ;
#10392=DIRECTION('ref_axis',(0.877582561890372,-0.479425538604204,0.)) ;
#10393=DIRECTION('center_axis',(0.479425538604204,0.877582561890372,0.)) ;
#10394=DIRECTION('ref_axis',(-0.877582561890372,0.479425538604204,0.)) ;
#10395=DIRECTION('center_axis',(0.,0.,-1.)) ;
#10396=DIRECTION('ref_axis',(1.,0.,0.)) ;
#10397=DIRECTION('center_axis',(0.,0.,1.)) ;
#10398=DIRECTION('ref_axis',(0.877582561890372,-0.479425538604204,0.)) ;
#10399=DIRECTION('center_axis',(0.,0.,1.)) ;
#10400=DIRECTION('ref_axis',(-1.,0.,0.)) ;
#10401=DIRECTION('',(0.824657857539967,-0.450512640843331,-0.342020143321939)) ;
#10402=DIRECTION('center_axis',(0.,0.,-1.)) ;
#10403=DIRECTION('ref_axis',(0.877582561890372,-0.479425538604204,0.)) ;
#10404=DIRECTION('center_axis',(-0.479425538604204,-0.877582561890372,0.)) ;
#10405=DIRECTION('ref_axis',(-0.877582561890372,0.479425538604204,0.)) ;
#10406=DIRECTION('center_axis',(0.,0.,-1.)) ;
#10407=DIRECTION('ref_axis',(1.,0.,0.)) ;
#10408=DIRECTION('center_axis',(0.,0.,-1.)) ;
#10409=DIRECTION('ref_axis',(0.877582561890372,-0.479425538604204,0.)) ;
#10410=DIRECTION('',(-0.864250110858646,0.472141987409852,-0.173648177662463)) ;
#10411=DIRECTION('center_axis',(0.,0.,-1.)) ;
#10412=DIRECTION('ref_axis',(1.,0.,0.)) ;
#10413=DIRECTION('center_axis',(0.,0.,1.)) ;
#10414=DIRECTION('ref_axis',(0.877582561890372,-0.479425538604204,0.)) ;
#10415=DIRECTION('center_axis',(0.,0.,1.)) ;
#10416=DIRECTION('ref_axis',(-1.,0.,0.)) ;
#10417=DIRECTION('',(0.152390612624165,-0.0832513711054022,-0.984807753012283)) ;
#10418=DIRECTION('center_axis',(0.,0.,-1.)) ;
#10419=DIRECTION('ref_axis',(0.877582561890373,-0.479425538604203,0.)) ;
#10420=DIRECTION('',(0.864250110858646,-0.47214198740985,0.173648177662463)) ;
#10421=DIRECTION('center_axis',(0.,0.,-1.)) ;
#10422=DIRECTION('ref_axis',(1.,0.,0.)) ;
#10423=DIRECTION('center_axis',(0.,0.,-1.)) ;
#10424=DIRECTION('ref_axis',(0.877582561890372,-0.479425538604204,0.)) ;
#10425=DIRECTION('center_axis',(0.479425538604204,0.877582561890372,0.)) ;
#10426=DIRECTION('ref_axis',(-0.877582561890372,0.479425538604204,0.)) ;
#10427=DIRECTION('center_axis',(0.,0.,-1.)) ;
#10428=DIRECTION('ref_axis',(1.,0.,0.)) ;
#10429=DIRECTION('center_axis',(0.,0.,1.)) ;
#10430=DIRECTION('ref_axis',(0.877582561890372,-0.479425538604204,0.)) ;
#10431=DIRECTION('center_axis',(0.,0.,1.)) ;
#10432=DIRECTION('ref_axis',(-1.,0.,0.)) ;
#10433=DIRECTION('',(-0.824657857539967,0.450512640843331,0.342020143321939)) ;
#10434=DIRECTION('center_axis',(0.,0.,-1.)) ;
#10435=DIRECTION('ref_axis',(0.877582561890372,-0.479425538604204,0.)) ;
#10436=DIRECTION('center_axis',(-0.479425538604204,-0.877582561890372,0.)) ;
#10437=DIRECTION('ref_axis',(-0.877582561890372,0.479425538604204,0.)) ;
#10438=DIRECTION('center_axis',(0.,0.,-1.)) ;
#10439=DIRECTION('ref_axis',(1.,0.,0.)) ;
#10440=DIRECTION('center_axis',(0.,0.,-1.)) ;
#10441=DIRECTION('ref_axis',(1.,0.,0.)) ;
#10442=DIRECTION('center_axis',(0.,0.,-1.)) ;
#10443=DIRECTION('ref_axis',(1.,0.,0.)) ;
#10444=DIRECTION('center_axis',(0.,0.,-1.)) ;
#10445=DIRECTION('ref_axis',(0.877582561890372,-0.479425538604204,0.)) ;
#10446=DIRECTION('center_axis',(-0.479425538604204,-0.877582561890372,0.)) ;
#10447=DIRECTION('ref_axis',(-0.877582561890372,0.479425538604204,0.)) ;
#10448=DIRECTION('center_axis',(0.,0.,-1.)) ;
#10449=DIRECTION('ref_axis',(1.,0.,0.)) ;
#10450=DIRECTION('center_axis',(0.,0.,-1.)) ;
#10451=DIRECTION('ref_axis',(0.877582561890372,-0.479425538604204,0.)) ;
#10452=DIRECTION('',(0.,0.,1.)) ;
#10453=DIRECTION('center_axis',(0.,0.,-1.)) ;
#10454=DIRECTION('ref_axis',(1.,0.,0.)) ;
#10455=DIRECTION('center_axis',(0.,0.,-1.)) ;
#10456=DIRECTION('ref_axis',(1.,0.,0.)) ;
#10457=DIRECTION('center_axis',(0.,0.,-1.)) ;
#10458=DIRECTION('ref_axis',(1.,0.,0.)) ;
#10459=DIRECTION('center_axis',(0.,0.,-1.)) ;
#10460=DIRECTION('ref_axis',(0.877582561890372,-0.479425538604204,0.)) ;
#10461=DIRECTION('center_axis',(0.,0.,-1.)) ;
#10462=DIRECTION('ref_axis',(1.,0.,0.)) ;
#10463=DIRECTION('center_axis',(0.479425538604204,0.877582561890372,0.)) ;
#10464=DIRECTION('ref_axis',(-0.877582561890372,0.479425538604204,0.)) ;
#10465=DIRECTION('center_axis',(0.,0.,-1.)) ;
#10466=DIRECTION('ref_axis',(1.,0.,0.)) ;
#10467=DIRECTION('center_axis',(0.,0.,-1.)) ;
#10468=DIRECTION('ref_axis',(0.877582561890372,-0.479425538604204,0.)) ;
#10469=DIRECTION('',(0.,0.,1.)) ;
#10470=DIRECTION('center_axis',(0.,0.,-1.)) ;
#10471=DIRECTION('ref_axis',(1.,0.,0.)) ;
#10472=DIRECTION('center_axis',(0.,0.,-1.)) ;
#10473=DIRECTION('ref_axis',(1.,0.,0.)) ;
#10474=DIRECTION('center_axis',(0.,0.,-1.)) ;
#10475=DIRECTION('ref_axis',(1.,0.,0.)) ;
#10476=DIRECTION('center_axis',(0.,0.,-1.)) ;
#10477=DIRECTION('ref_axis',(1.,0.,0.)) ;
#10478=DIRECTION('center_axis',(0.,0.,-1.)) ;
#10479=DIRECTION('ref_axis',(1.,0.,0.)) ;
#10480=DIRECTION('center_axis',(0.,0.,-1.)) ;
#10481=DIRECTION('ref_axis',(0.877582561890372,-0.479425538604204,0.)) ;
#10482=DIRECTION('center_axis',(0.,0.,-1.)) ;
#10483=DIRECTION('ref_axis',(1.,0.,0.)) ;
#10484=DIRECTION('center_axis',(0.479425538604204,0.877582561890372,0.)) ;
#10485=DIRECTION('ref_axis',(-0.877582561890372,0.479425538604204,0.)) ;
#10486=DIRECTION('center_axis',(0.,0.,-1.)) ;
#10487=DIRECTION('ref_axis',(0.877582561890372,-0.479425538604204,0.)) ;
#10488=DIRECTION('center_axis',(0.479425538604204,0.877582561890372,0.)) ;
#10489=DIRECTION('ref_axis',(-0.877582561890372,0.479425538604204,0.)) ;
#10490=DIRECTION('center_axis',(0.,0.,-1.)) ;
#10491=DIRECTION('ref_axis',(1.,0.,0.)) ;
#10492=DIRECTION('center_axis',(0.,0.,-1.)) ;
#10493=DIRECTION('ref_axis',(0.877582561890372,-0.479425538604204,0.)) ;
#10494=DIRECTION('center_axis',(0.,0.,-1.)) ;
#10495=DIRECTION('ref_axis',(1.,0.,0.)) ;
#10496=DIRECTION('',(0.824657857539967,-0.450512640843331,0.342020143321939)) ;
#10497=DIRECTION('center_axis',(0.,0.,-1.)) ;
#10498=DIRECTION('ref_axis',(0.877582561890372,-0.479425538604204,0.)) ;
#10499=DIRECTION('',(0.,0.,-1.)) ;
#10500=DIRECTION('center_axis',(0.,0.,-1.)) ;
#10501=DIRECTION('ref_axis',(1.,0.,0.)) ;
#10502=DIRECTION('center_axis',(0.,0.,-1.)) ;
#10503=DIRECTION('ref_axis',(0.877582561890372,-0.479425538604204,0.)) ;
#10504=DIRECTION('center_axis',(0.,0.,-1.)) ;
#10505=DIRECTION('ref_axis',(1.,0.,0.)) ;
#10506=DIRECTION('center_axis',(-0.479425538604204,-0.877582561890372,0.)) ;
#10507=DIRECTION('ref_axis',(-0.877582561890372,0.479425538604204,0.)) ;
#10508=DIRECTION('center_axis',(0.,0.,-1.)) ;
#10509=DIRECTION('ref_axis',(0.877582561890372,-0.479425538604204,0.)) ;
#10510=DIRECTION('center_axis',(0.479425538604204,0.877582561890372,0.)) ;
#10511=DIRECTION('ref_axis',(-0.877582561890372,0.479425538604204,0.)) ;
#10512=DIRECTION('center_axis',(0.,0.,-1.)) ;
#10513=DIRECTION('ref_axis',(1.,0.,0.)) ;
#10514=DIRECTION('center_axis',(0.,0.,1.)) ;
#10515=DIRECTION('ref_axis',(0.877582561890372,-0.479425538604204,0.)) ;
#10516=DIRECTION('',(-0.864250110858646,0.472141987409852,0.173648177662463)) ;
#10517=DIRECTION('center_axis',(0.,0.,1.)) ;
#10518=DIRECTION('ref_axis',(-1.,0.,0.)) ;
#10519=DIRECTION('center_axis',(0.,0.,-1.)) ;
#10520=DIRECTION('ref_axis',(1.,0.,0.)) ;
#10521=DIRECTION('center_axis',(0.,0.,-1.)) ;
#10522=DIRECTION('ref_axis',(1.,0.,0.)) ;
#10523=DIRECTION('center_axis',(0.,0.,-1.)) ;
#10524=DIRECTION('ref_axis',(0.877582561890372,-0.479425538604204,0.)) ;
#10525=DIRECTION('center_axis',(0.,0.,-1.)) ;
#10526=DIRECTION('ref_axis',(1.,0.,0.)) ;
#10527=DIRECTION('',(0.152390612624165,-0.0832513711054022,0.984807753012283)) ;
#10528=DIRECTION('center_axis',(0.,0.,-1.)) ;
#10529=DIRECTION('ref_axis',(0.877582561890372,-0.479425538604204,0.)) ;
#10530=DIRECTION('',(0.,0.,1.)) ;
#10531=DIRECTION('center_axis',(0.,0.,1.)) ;
#10532=DIRECTION('ref_axis',(0.877582561890373,-0.479425538604203,0.)) ;
#10533=DIRECTION('',(0.864250110858646,-0.47214198740985,-0.173648177662463)) ;
#10534=DIRECTION('center_axis',(0.,0.,1.)) ;
#10535=DIRECTION('ref_axis',(-1.,0.,0.)) ;
#10536=DIRECTION('center_axis',(0.,0.,-1.)) ;
#10537=DIRECTION('ref_axis',(0.877582561890372,-0.479425538604204,0.)) ;
#10538=DIRECTION('center_axis',(0.,0.,-1.)) ;
#10539=DIRECTION('ref_axis',(1.,0.,0.)) ;
#10540=DIRECTION('center_axis',(0.479425538604204,0.877582561890372,0.)) ;
#10541=DIRECTION('ref_axis',(-0.877582561890372,0.479425538604204,0.)) ;
#10542=DIRECTION('center_axis',(0.,0.,-1.)) ;
#10543=DIRECTION('ref_axis',(0.877582561890372,-0.479425538604204,0.)) ;
#10544=DIRECTION('center_axis',(0.,0.,-1.)) ;
#10545=DIRECTION('ref_axis',(1.,0.,0.)) ;
#10546=DIRECTION('',(-0.824657857539967,0.450512640843331,-0.342020143321939)) ;
#10547=DIRECTION('center_axis',(0.,0.,-1.)) ;
#10548=DIRECTION('ref_axis',(0.877582561890372,-0.479425538604204,0.)) ;
#10549=DIRECTION('center_axis',(0.,0.,-1.)) ;
#10550=DIRECTION('ref_axis',(1.,0.,0.)) ;
#10551=DIRECTION('center_axis',(-0.479425538604204,-0.877582561890372,0.)) ;
#10552=DIRECTION('ref_axis',(-0.877582561890372,0.479425538604204,0.)) ;
#10553=DIRECTION('center_axis',(0.,0.,-1.)) ;
#10554=DIRECTION('ref_axis',(1.,0.,0.)) ;
#10555=DIRECTION('center_axis',(0.,0.,-1.)) ;
#10556=DIRECTION('ref_axis',(1.,0.,0.)) ;
#10557=DIRECTION('center_axis',(0.,0.,-1.)) ;
#10558=DIRECTION('ref_axis',(0.877582561890372,-0.479425538604204,0.)) ;
#10559=DIRECTION('center_axis',(0.,0.,-1.)) ;
#10560=DIRECTION('ref_axis',(1.,0.,0.)) ;
#10561=DIRECTION('center_axis',(-0.479425538604204,-0.877582561890372,0.)) ;
#10562=DIRECTION('ref_axis',(-0.877582561890372,0.479425538604204,0.)) ;
#10563=DIRECTION('center_axis',(0.,0.,-1.)) ;
#10564=DIRECTION('ref_axis',(0.877582561890372,-0.479425538604204,0.)) ;
#10565=DIRECTION('center_axis',(0.,0.,-1.)) ;
#10566=DIRECTION('ref_axis',(1.,0.,0.)) ;
#10567=DIRECTION('',(0.,0.,1.)) ;
#10568=DIRECTION('center_axis',(0.,0.,-1.)) ;
#10569=DIRECTION('ref_axis',(1.,0.,0.)) ;
#10570=DIRECTION('center_axis',(0.,0.,-1.)) ;
#10571=DIRECTION('ref_axis',(1.,0.,0.)) ;
#10572=DIRECTION('center_axis',(0.,0.,-1.)) ;
#10573=DIRECTION('ref_axis',(0.877582561890372,-0.479425538604204,0.)) ;
#10574=DIRECTION('center_axis',(0.,0.,-1.)) ;
#10575=DIRECTION('ref_axis',(1.,0.,0.)) ;
#10576=DIRECTION('',(0.,0.,1.)) ;
#10577=DIRECTION('center_axis',(0.,0.,-1.)) ;
#10578=DIRECTION('ref_axis',(0.877582561890372,-0.479425538604204,0.)) ;
#10579=DIRECTION('center_axis',(0.,0.,-1.)) ;
#10580=DIRECTION('ref_axis',(1.,0.,0.)) ;
#10581=DIRECTION('center_axis',(-0.479425538604204,-0.877582561890372,0.)) ;
#10582=DIRECTION('ref_axis',(-0.877582561890372,0.479425538604204,0.)) ;
#10583=DIRECTION('center_axis',(0.,0.,-1.)) ;
#10584=DIRECTION('ref_axis',(0.877582561890372,-0.479425538604204,0.)) ;
#10585=DIRECTION('',(0.,0.,1.)) ;
#12968=CARTESIAN_POINT('',(0.,0.,0.)) ;
#12969=CARTESIAN_POINT('Origin',(0.,0.,3.4)) ;
#12970=CARTESIAN_POINT('',(-8.24927608177,4.50660006288,3.4)) ;
#12971=CARTESIAN_POINT('Origin',(0.,0.,3.4)) ;
#12972=CARTESIAN_POINT('',(-8.38091346605,4.57851389367,3.25)) ;
#12973=CARTESIAN_POINT('Origin',(-8.38091346605305,4.57851389367015,3.4)) ;
#12974=CARTESIAN_POINT('Origin',(0.,0.,3.25)) ;
#12975=CARTESIAN_POINT('Origin',(11.3794692077,0.,3.25)) ;
#12976=CARTESIAN_POINT('',(-9.98642374024597,5.45560815393152,3.25)) ;
#12977=CARTESIAN_POINT('Origin',(0.,0.,3.25)) ;
#12978=CARTESIAN_POINT('Origin',(0.,0.,3.7)) ;
#12979=CARTESIAN_POINT('',(-10.121491651368,5.5293960900755,3.27713832065)) ;
#12980=CARTESIAN_POINT('Origin',(-9.98642374024597,5.45560815393153,3.7)) ;
#12981=CARTESIAN_POINT('Origin',(0.,0.,3.27713832065)) ;
#12982=CARTESIAN_POINT('Origin',(0.,0.,3.27713832065)) ;
#12983=CARTESIAN_POINT('',(-10.2861369405,5.61934222145,3.345423616)) ;
#12984=CARTESIAN_POINT('Origin',(0.,0.,3.345423616)) ;
#12985=CARTESIAN_POINT('',(-10.121491651368,5.52939609007551,3.27713832065)) ;
#12986=CARTESIAN_POINT('Origin',(0.,0.,3.01653119873)) ;
#12987=CARTESIAN_POINT('',(-10.4445264746,5.70587081833,3.36121391227)) ;
#12988=CARTESIAN_POINT('Origin',(-10.3911897601781,5.67673283842462,3.01653119873)) ;
#12989=CARTESIAN_POINT('Origin',(0.,0.,3.36121391227)) ;
#12990=CARTESIAN_POINT('Origin',(0.,0.,3.36121391228)) ;
#12991=CARTESIAN_POINT('',(-11.1802248884,6.10778469353,3.21339479458)) ;
#12992=CARTESIAN_POINT('',(-10.4445264746112,5.70587081831953,3.36121391228)) ;
#12993=CARTESIAN_POINT('Origin',(0.,0.,3.21339479458)) ;
#12994=CARTESIAN_POINT('Origin',(0.,0.,3.21339479458)) ;
#12995=CARTESIAN_POINT('',(-11.1954639496152,6.11610983063119,3.31187556988574)) ;
#12996=CARTESIAN_POINT('Origin',(0.,0.,3.31187556988)) ;
#12997=CARTESIAN_POINT('',(-11.1802248883521,6.10778469352028,3.21339479458)) ;
#12998=CARTESIAN_POINT('Origin',(0.,0.,3.45969468758)) ;
#12999=CARTESIAN_POINT('',(-10.4597655359029,5.71419595544604,3.45969468758)) ;
#13000=CARTESIAN_POINT('',(-10.4597655359029,5.71419595544604,3.45969468758)) ;
#13001=CARTESIAN_POINT('Origin',(0.,0.,3.45969468758)) ;
#13002=CARTESIAN_POINT('Origin',(0.,0.,3.01653119873)) ;
#13003=CARTESIAN_POINT('',(-10.2561218490561,5.60294490228063,3.43939287808)) ;
#13004=CARTESIAN_POINT('Origin',(-10.3911897601781,5.67673283842462,3.01653119873)) ;
#13005=CARTESIAN_POINT('Origin',(0.,0.,3.43939287808)) ;
#13006=CARTESIAN_POINT('Origin',(0.,0.,3.37110758272)) ;
#13007=CARTESIAN_POINT('',(-10.0914765600368,5.51299877094837,3.37110758272)) ;
#13008=CARTESIAN_POINT('Origin',(0.,0.,3.37110758272)) ;
#13009=CARTESIAN_POINT('',(-10.0914765600368,5.51299877094838,3.37110758272)) ;
#13010=CARTESIAN_POINT('Origin',(0.,0.,3.7)) ;
#13011=CARTESIAN_POINT('',(-9.98642374026,5.45560815394,3.35)) ;
#13012=CARTESIAN_POINT('Origin',(-9.98642374024597,5.45560815393153,3.7)) ;
#13013=CARTESIAN_POINT('Origin',(0.,0.,3.35)) ;
#13014=CARTESIAN_POINT('Origin',(11.3794692077,0.,3.35)) ;
#13015=CARTESIAN_POINT('',(-8.38091346605306,4.57851389367014,3.35)) ;
#13016=CARTESIAN_POINT('Origin',(0.,0.,3.35)) ;
#13017=CARTESIAN_POINT('Origin',(0.,0.,3.4)) ;
#13018=CARTESIAN_POINT('',(-8.33703433795854,4.55454261673993,3.4)) ;
#13019=CARTESIAN_POINT('Origin',(-8.38091346605305,4.57851389367015,3.4)) ;
#13020=CARTESIAN_POINT('Origin',(0.,0.,3.4)) ;
#13021=CARTESIAN_POINT('Origin',(0.,0.,9.46868240833)) ;
#13022=CARTESIAN_POINT('',(-8.33703433796,4.55454261674,3.8)) ;
#13023=CARTESIAN_POINT('',(-8.33703433795854,4.55454261673994,9.46868240833)) ;
#13024=CARTESIAN_POINT('Origin',(0.,0.,3.8)) ;
#13025=CARTESIAN_POINT('Origin',(9.5,0.,3.8)) ;
#13026=CARTESIAN_POINT('',(-8.24927608177,4.50660006288,3.8)) ;
#13027=CARTESIAN_POINT('Origin',(0.,0.,3.8)) ;
#13028=CARTESIAN_POINT('Origin',(0.,0.,9.6)) ;
#13029=CARTESIAN_POINT('',(-8.38091346605306,4.57851389367015,9.75)) ;
#13030=CARTESIAN_POINT('Origin',(0.,0.,9.75)) ;
#13031=CARTESIAN_POINT('',(-8.2492760817695,4.50660006287951,9.6)) ;
#13032=CARTESIAN_POINT('Origin',(-8.38091346605305,4.57851389367015,9.6)) ;
#13033=CARTESIAN_POINT('Origin',(0.,0.,9.6)) ;
#13034=CARTESIAN_POINT('Origin',(0.,0.,6.50000000002)) ;
#13035=CARTESIAN_POINT('',(-8.24927608177,4.50660006288,10.)) ;
#13036=CARTESIAN_POINT('',(-8.2492760817695,4.50660006287952,6.50000000002)) ;
#13037=CARTESIAN_POINT('Origin',(0.,0.,10.)) ;
#13038=CARTESIAN_POINT('Origin',(11.3794692077,0.,9.75)) ;
#13039=CARTESIAN_POINT('',(-9.98642374026,5.45560815394,9.75)) ;
#13040=CARTESIAN_POINT('Origin',(0.,0.,9.75)) ;
#13041=CARTESIAN_POINT('Origin',(7.8,0.,10.)) ;
#13042=CARTESIAN_POINT('',(-6.84514398274491,3.73951920111279,10.)) ;
#13043=CARTESIAN_POINT('Origin',(0.,0.,10.)) ;
#13044=CARTESIAN_POINT('Origin',(0.,0.,9.3)) ;
#13045=CARTESIAN_POINT('',(-10.1214916514,5.52939609008,9.72286167935)) ;
#13046=CARTESIAN_POINT('Origin',(0.,0.,9.72286167935)) ;
#13047=CARTESIAN_POINT('Origin',(-9.98642374024597,5.45560815393153,9.3)) ;
#13048=CARTESIAN_POINT('Origin',(0.,0.,9.7)) ;
#13049=CARTESIAN_POINT('',(-6.58186921417779,3.59569153953153,9.7)) ;
#13050=CARTESIAN_POINT('Origin',(-6.8451439827449,3.73951920111279,9.7)) ;
#13051=CARTESIAN_POINT('Origin',(0.,0.,9.7)) ;
#13052=CARTESIAN_POINT('Origin',(0.,0.,9.72286167935)) ;
#13053=CARTESIAN_POINT('',(-10.2861369404706,5.6193422214533,9.65457638398625)) ;
#13054=CARTESIAN_POINT('Origin',(0.,0.,9.654576384)) ;
#13055=CARTESIAN_POINT('',(-10.121491651368,5.52939609007551,9.72286167935)) ;
#13056=CARTESIAN_POINT('Origin',(0.,0.,6.50000000002)) ;
#13057=CARTESIAN_POINT('',(-6.58186921417779,3.59569153953153,3.3)) ;
#13058=CARTESIAN_POINT('',(-6.58186921417779,3.59569153953153,6.50000000002)) ;
#13059=CARTESIAN_POINT('Origin',(0.,0.,3.3)) ;
#13060=CARTESIAN_POINT('Origin',(0.,0.,9.98346880127)) ;
#13061=CARTESIAN_POINT('',(-10.4445264746112,5.70587081831952,9.63878608773)) ;
#13062=CARTESIAN_POINT('Origin',(0.,0.,9.63878608773)) ;
#13063=CARTESIAN_POINT('Origin',(-10.3911897601781,5.67673283842462,9.98346880127)) ;
#13064=CARTESIAN_POINT('Origin',(0.,0.,3.3)) ;
#13065=CARTESIAN_POINT('',(-6.84514398274491,3.73951920111279,3.)) ;
#13066=CARTESIAN_POINT('Origin',(-6.8451439827449,3.73951920111279,3.3)) ;
#13067=CARTESIAN_POINT('Origin',(0.,0.,3.)) ;
#13068=CARTESIAN_POINT('Origin',(0.,0.,9.63878608772)) ;
#13069=CARTESIAN_POINT('',(-11.1802248883528,6.10778469352065,9.78660520541552)) ;
#13070=CARTESIAN_POINT('',(-10.4445264746112,5.70587081831953,9.63878608772)) ;
#13071=CARTESIAN_POINT('Origin',(0.,0.,9.78660520542)) ;
#13072=CARTESIAN_POINT('Origin',(7.8,0.,3.)) ;
#13073=CARTESIAN_POINT('',(-8.24927608177,4.50660006288,3.)) ;
#13074=CARTESIAN_POINT('Origin',(0.,0.,3.)) ;
#13075=CARTESIAN_POINT('Origin',(0.,0.,9.78660520542)) ;
#13076=CARTESIAN_POINT('',(-11.1954639496,6.11610983064,9.68812443012)) ;
#13077=CARTESIAN_POINT('Origin',(0.,0.,9.68812443012)) ;
#13078=CARTESIAN_POINT('',(-11.1802248883521,6.10778469352028,9.78660520542)) ;
#13079=CARTESIAN_POINT('Origin',(0.,0.,6.50000000002)) ;
#13080=CARTESIAN_POINT('',(-8.2492760817695,4.50660006287952,6.50000000002)) ;
#13081=CARTESIAN_POINT('Origin',(0.,0.,9.54030531242)) ;
#13082=CARTESIAN_POINT('',(-10.4597655359,5.71419595544,9.54030531242)) ;
#13083=CARTESIAN_POINT('',(-10.4597655359029,5.71419595544604,9.54030531242)) ;
#13084=CARTESIAN_POINT('Origin',(0.,0.,9.54030531242)) ;
#13085=CARTESIAN_POINT('Origin',(0.,0.,9.98346880127)) ;
#13086=CARTESIAN_POINT('',(-10.2561218491,5.6029449023,9.56060712192)) ;
#13087=CARTESIAN_POINT('Origin',(0.,0.,9.56060712192)) ;
#13088=CARTESIAN_POINT('Origin',(-10.3911897601781,5.67673283842462,9.98346880127)) ;
#13089=CARTESIAN_POINT('Origin',(0.,0.,9.62889241728)) ;
#13090=CARTESIAN_POINT('',(-10.09147656,5.51299877094,9.62889241728)) ;
#13091=CARTESIAN_POINT('Origin',(0.,0.,9.62889241728)) ;
#13092=CARTESIAN_POINT('',(-10.0914765600368,5.51299877094839,9.62889241728)) ;
#13093=CARTESIAN_POINT('Origin',(0.,0.,9.3)) ;
#13094=CARTESIAN_POINT('',(-9.98642374024597,5.45560815393152,9.65)) ;
#13095=CARTESIAN_POINT('Origin',(0.,0.,9.65)) ;
#13096=CARTESIAN_POINT('Origin',(-9.98642374024597,5.45560815393153,9.3)) ;
#13097=CARTESIAN_POINT('Origin',(11.3794692077,0.,9.65)) ;
#13098=CARTESIAN_POINT('',(-8.38091346605,4.57851389367,9.65)) ;
#13099=CARTESIAN_POINT('Origin',(0.,0.,9.65)) ;
#13100=CARTESIAN_POINT('Origin',(0.,0.,9.6)) ;
#13101=CARTESIAN_POINT('',(-8.33703433796,4.55454261674,9.6)) ;
#13102=CARTESIAN_POINT('Origin',(0.,0.,9.6)) ;
#13103=CARTESIAN_POINT('Origin',(-8.38091346605305,4.57851389367015,9.6)) ;
#13104=CARTESIAN_POINT('Origin',(0.,0.,9.46868240833)) ;
#13105=CARTESIAN_POINT('',(-8.33703433795854,4.55454261673994,9.2)) ;
#13106=CARTESIAN_POINT('Origin',(0.,0.,9.2)) ;
#13107=CARTESIAN_POINT('',(-8.33703433795854,4.55454261673994,9.46868240833)) ;
#13108=CARTESIAN_POINT('Origin',(9.5,0.,9.2)) ;
#13109=CARTESIAN_POINT('',(-8.2492760817695,4.50660006287951,9.2)) ;
#13110=CARTESIAN_POINT('Origin',(0.,0.,9.2)) ;
#13111=CARTESIAN_POINT('Origin',(0.,0.,6.50000000002)) ;
#13112=CARTESIAN_POINT('',(-8.2492760817695,4.50660006287951,7.95524052995)) ;
#13113=CARTESIAN_POINT('Origin',(0.,0.,7.95524052995)) ;
#13114=CARTESIAN_POINT('',(-8.2492760817695,4.50660006287952,6.50000000002)) ;
#13115=CARTESIAN_POINT('Origin',(0.,0.,6.5)) ;
#13116=CARTESIAN_POINT('',(-8.24927608177,4.50660006288,5.04475947005)) ;
#13117=CARTESIAN_POINT('Origin',(0.,0.,5.04475947005)) ;
#13118=CARTESIAN_POINT('Origin',(-9.4340125403215,5.15382453999519,6.5)) ;
#13119=CARTESIAN_POINT('Origin',(0.,0.,6.50000000002)) ;
#13120=CARTESIAN_POINT('',(-8.2492760817695,4.50660006287952,6.50000000002)) ;
#13487=UNCERTAINTY_MEASURE_WITH_UNIT(LENGTH_MEASURE(0.01),#13511,
'DISTANCE_ACCURACY_VALUE',
'Maximum model space distance between geometric entities at asserted c
onnectivities') ;
#13493=UNCERTAINTY_MEASURE_WITH_UNIT(LENGTH_MEASURE(0.01),#13511,
'DISTANCE_ACCURACY_VALUE',
'Maximum model space distance between geometric entities at asserted c
onnectivities') ;
#13504=(
GEOMETRIC_REPRESENTATION_CONTEXT(3)
GLOBAL_UNCERTAINTY_ASSIGNED_CONTEXT((#13487))
GLOBAL_UNIT_ASSIGNED_CONTEXT((#13511,#13513,#13514))
REPRESENTATION_CONTEXT('','3D')
) ;
#13510=(
GEOMETRIC_REPRESENTATION_CONTEXT(3)
GLOBAL_UNCERTAINTY_ASSIGNED_CONTEXT((#13493))
GLOBAL_UNIT_ASSIGNED_CONTEXT((#13511,#13513,#13514))
REPRESENTATION_CONTEXT('','3D')
) ;
#13511=(
LENGTH_UNIT()
NAMED_UNIT(*)
SI_UNIT(.MILLI.,.METRE.)
) ;
#13513=(
NAMED_UNIT(*)
PLANE_ANGLE_UNIT()
SI_UNIT($,.RADIAN.)
) ;
#13514=(
NAMED_UNIT(*)
SI_UNIT($,.STERADIAN.)
SOLID_ANGLE_UNIT()
) ;
#13525=SHAPE_DEFINITION_REPRESENTATION(#13541,#13572) ;
#13541=PRODUCT_DEFINITION_SHAPE('',$,#13589) ;
#13572=SHAPE_REPRESENTATION('',(#8252),#13504) ;
#13578=PRODUCT_DEFINITION_CONTEXT('part definition',#13628,'design') ;
#13589=PRODUCT_DEFINITION('Front_Bearing_Race','Front_Bearing_Race',#13605,
#13578) ;
#13605=PRODUCT_DEFINITION_FORMATION('',$,#13640) ;
#13628=APPLICATION_CONTEXT(
'Core Data for Automotive Mechanical Design Process') ;
#13629=PRODUCT_CONTEXT('part definition',#13628,'mechanical') ;
#13640=PRODUCT('Front_Bearing_Race','Front_Bearing_Race',$,(#13629)) ;
#13650=PRESENTATION_STYLE_ASSIGNMENT((#13655)) ;
#13655=SURFACE_STYLE_USAGE(.BOTH.,#13660) ;
#13660=SURFACE_SIDE_STYLE('',(#13665)) ;
#13665=SURFACE_STYLE_FILL_AREA(#13670) ;
#13670=FILL_AREA_STYLE('Opaque(144,144,144)',(#13675)) ;
#13675=FILL_AREA_STYLE_COLOUR('Opaque(144,144,144)',#13680) ;
#13680=COLOUR_RGB('Opaque(144,144,144)', 0.40784314, 0.44705882, 0.49803922) ;
ENDSEC;
END-ISO-10303-21;
